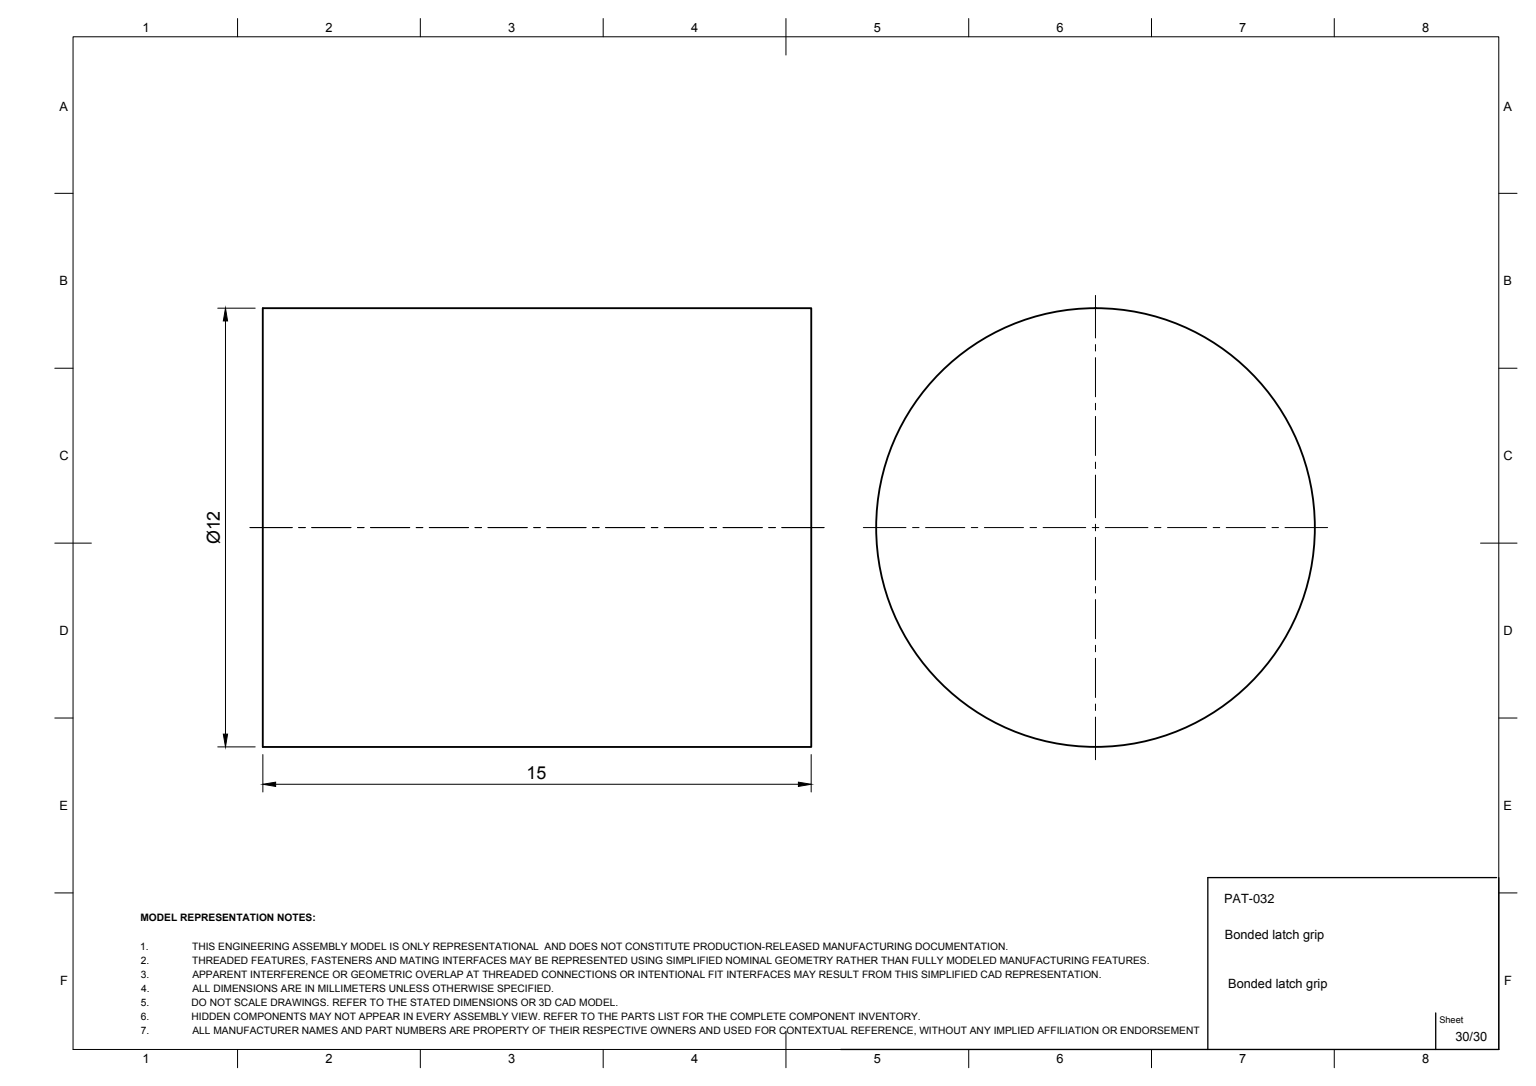
ISO-10303-21;
HEADER;
/* Generated by software containing ST-Developer
 * from STEP Tools, Inc. (www.steptools.com) 
 */

FILE_DESCRIPTION(
/* description */ ('Drill jig with bushing plate'),
/* implementation_level */ '2;1');

FILE_NAME(
/* name */ 'Bonded latch grip.step',
/* time_stamp */ '2026-10-27T10:51:08-07:00',
/* author */ (''),
/* organization */ (''),
/* preprocessor_version */ 'ST-DEVELOPER v20.2',
/* originating_system */ 'Autodesk Translation Framework v15.17.0.0',
/* authorisation */ '');

FILE_SCHEMA (('AUTOMOTIVE_DESIGN { 1 0 10303 214 3 1 1 }'));
ENDSEC;

DATA;
#10=MECHANICAL_DESIGN_GEOMETRIC_PRESENTATION_REPRESENTATION('',(#246),#6638);
#198=SHAPE_REPRESENTATION_RELATIONSHIP('SRR','None',#6764,#222);
#222=ADVANCED_BREP_SHAPE_REPRESENTATION('',(#268),#6637);
#246=STYLED_ITEM('',(#6950),#268);
#268=MANIFOLD_SOLID_BREP('Body1',#3615);
#499=PLANE('',#4322);
#500=PLANE('',#4323);
#712=FACE_OUTER_BOUND('',#1027,.T.);
#713=FACE_OUTER_BOUND('',#1028,.T.);
#714=FACE_OUTER_BOUND('',#1029,.T.);
#1027=EDGE_LOOP('',(#3293,#3294,#3295,#3296));
#1028=EDGE_LOOP('',(#3297));
#1029=EDGE_LOOP('',(#3298));
#1290=LINE('',#6572,#1551);
#1551=VECTOR('',#5469,0.6);
#1718=CIRCLE('',#4320,0.6);
#1719=CIRCLE('',#4321,0.6);
#2004=VERTEX_POINT('',#6569);
#2005=VERTEX_POINT('',#6571);
#2434=EDGE_CURVE('',#2004,#2004,#1718,.T.);
#2435=EDGE_CURVE('',#2004,#2005,#1290,.T.);
#2436=EDGE_CURVE('',#2005,#2005,#1719,.T.);
#3293=ORIENTED_EDGE('',*,*,#2434,.F.);
#3294=ORIENTED_EDGE('',*,*,#2435,.T.);
#3295=ORIENTED_EDGE('',*,*,#2436,.T.);
#3296=ORIENTED_EDGE('',*,*,#2435,.F.);
#3297=ORIENTED_EDGE('',*,*,#2434,.T.);
#3298=ORIENTED_EDGE('',*,*,#2436,.F.);
#3375=CYLINDRICAL_SURFACE('',#4319,0.6);
#3587=ADVANCED_FACE('',(#712),#3375,.T.);
#3588=ADVANCED_FACE('',(#713),#499,.T.);
#3589=ADVANCED_FACE('',(#714),#500,.F.);
#3615=CLOSED_SHELL('',(#3587,#3588,#3589));
#4318=AXIS2_PLACEMENT_3D('',#6567,#5463,#5464);
#4319=AXIS2_PLACEMENT_3D('',#6568,#5465,#5466);
#4320=AXIS2_PLACEMENT_3D('',#6570,#5467,#5468);
#4321=AXIS2_PLACEMENT_3D('',#6573,#5470,#5471);
#4322=AXIS2_PLACEMENT_3D('',#6574,#5472,#5473);
#4323=AXIS2_PLACEMENT_3D('',#6575,#5474,#5475);
#5463=DIRECTION('axis',(0.,0.,1.));
#5464=DIRECTION('refdir',(1.,0.,0.));
#5465=DIRECTION('center_axis',(0.,0.,1.));
#5466=DIRECTION('ref_axis',(1.,0.,0.));
#5467=DIRECTION('center_axis',(0.,0.,1.));
#5468=DIRECTION('ref_axis',(1.,0.,0.));
#5469=DIRECTION('',(0.,0.,-1.));
#5470=DIRECTION('center_axis',(0.,0.,1.));
#5471=DIRECTION('ref_axis',(1.,0.,0.));
#5472=DIRECTION('center_axis',(0.,0.,1.));
#5473=DIRECTION('ref_axis',(1.,0.,0.));
#5474=DIRECTION('center_axis',(0.,0.,1.));
#5475=DIRECTION('ref_axis',(1.,0.,0.));
#6567=CARTESIAN_POINT('',(0.,0.,0.));
#6568=CARTESIAN_POINT('Origin',(9.2,7.5,4.8));
#6569=CARTESIAN_POINT('',(8.6,7.5,6.3));
#6570=CARTESIAN_POINT('Origin',(9.2,7.5,6.3));
#6571=CARTESIAN_POINT('',(8.6,7.5,4.8));
#6572=CARTESIAN_POINT('',(8.6,7.5,4.8));
#6573=CARTESIAN_POINT('Origin',(9.2,7.5,4.8));
#6574=CARTESIAN_POINT('Origin',(9.2,7.5,6.3));
#6575=CARTESIAN_POINT('Origin',(9.2,7.5,4.8));
#6608=UNCERTAINTY_MEASURE_WITH_UNIT(LENGTH_MEASURE(0.001),#6639,
'DISTANCE_ACCURACY_VALUE',
'Maximum model space distance between geometric entities at asserted c
onnectivities');
#6609=UNCERTAINTY_MEASURE_WITH_UNIT(LENGTH_MEASURE(0.001),#6639,
'DISTANCE_ACCURACY_VALUE',
'Maximum model space distance between geometric entities at asserted c
onnectivities');
#6637=(
GEOMETRIC_REPRESENTATION_CONTEXT(3)
GLOBAL_UNCERTAINTY_ASSIGNED_CONTEXT((#6608))
GLOBAL_UNIT_ASSIGNED_CONTEXT((#6639,#6641,#6642))
REPRESENTATION_CONTEXT('','3D')
);
#6638=(
GEOMETRIC_REPRESENTATION_CONTEXT(3)
GLOBAL_UNCERTAINTY_ASSIGNED_CONTEXT((#6609))
GLOBAL_UNIT_ASSIGNED_CONTEXT((#6639,#6641,#6642))
REPRESENTATION_CONTEXT('','3D')
);
#6639=(
LENGTH_UNIT()
NAMED_UNIT(*)
SI_UNIT(.CENTI.,.METRE.)
);
#6641=(
NAMED_UNIT(*)
PLANE_ANGLE_UNIT()
SI_UNIT($,.RADIAN.)
);
#6642=(
NAMED_UNIT(*)
SI_UNIT($,.STERADIAN.)
SOLID_ANGLE_UNIT()
);
#6670=SHAPE_DEFINITION_REPRESENTATION(#6731,#6764);
#6731=PRODUCT_DEFINITION_SHAPE('',$,#6793);
#6764=SHAPE_REPRESENTATION('',(#4318),#6637);
#6765=PRODUCT_DEFINITION_CONTEXT('part definition',#6851,'design');
#6793=PRODUCT_DEFINITION('Bonded latch grip','Bonded latch grip',#6821,
#6765);
#6821=PRODUCT_DEFINITION_FORMATION('',$,#6880);
#6851=APPLICATION_CONTEXT(
'Core Data for Automotive Mechanical Design Process');
#6852=PRODUCT_CONTEXT('part definition',#6851,'mechanical');
#6880=PRODUCT('Bonded latch grip','Bonded latch grip',
'Bonded latch grip',(#6852));
#6944=COLOUR_RGB('Black',0.12,0.14,0.17);
#6945=FILL_AREA_STYLE_COLOUR('',#6944);
#6946=FILL_AREA_STYLE('',(#6945));
#6947=SURFACE_STYLE_FILL_AREA(#6946);
#6948=SURFACE_SIDE_STYLE('',(#6947));
#6949=SURFACE_STYLE_USAGE(.BOTH.,#6948);
#6950=PRESENTATION_STYLE_ASSIGNMENT((#6949));
ENDSEC;
END-ISO-10303-21;
